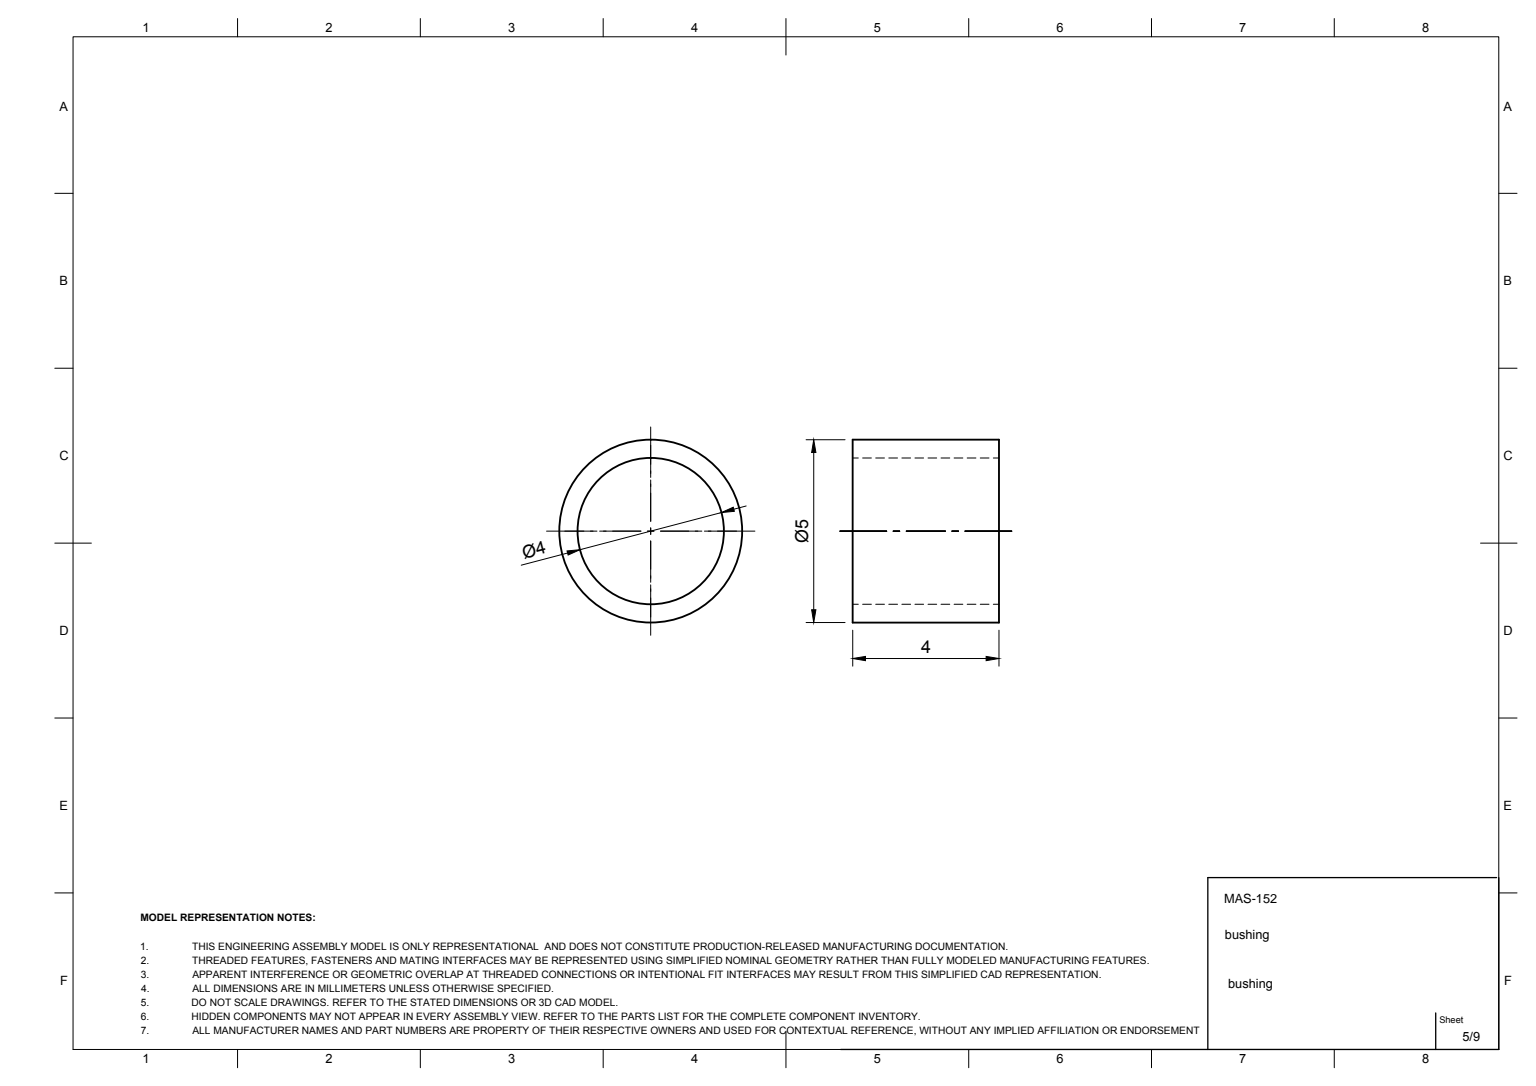
ISO-10303-21;
HEADER;
/* Generated by software containing ST-Developer
 * from STEP Tools, Inc. (www.steptools.com) 
 */

FILE_DESCRIPTION(
/* description */ ('STEP AP214'),
/* implementation_level */ '2;1');

FILE_NAME(
/* name */ 'bushing.step',
/* time_stamp */ '2026-11-04T19:18:53-08:00',
/* author */ (''),
/* organization */ (''),
/* preprocessor_version */ 'ST-DEVELOPER v20.2',
/* originating_system */ 'Autodesk Translation Framework v15.17.0.0',
/* authorisation */ '');

FILE_SCHEMA (('AUTOMOTIVE_DESIGN { 1 0 10303 214 3 1 1 }'));
ENDSEC;

DATA;
#10=MECHANICAL_DESIGN_GEOMETRIC_PRESENTATION_REPRESENTATION('',(#78),#5942);
#64=SHAPE_REPRESENTATION_RELATIONSHIP('SRR','None',#5975,#71);
#71=ADVANCED_BREP_SHAPE_REPRESENTATION('',(#85),#5935);
#78=STYLED_ITEM('',(#6019),#85);
#85=MANIFOLD_SOLID_BREP('Body1',#925);
#92=FACE_BOUND('',#197,.T.);
#93=FACE_BOUND('',#199,.T.);
#100=PLANE('',#1018);
#101=PLANE('',#1019);
#140=FACE_OUTER_BOUND('',#194,.T.);
#141=FACE_OUTER_BOUND('',#195,.T.);
#142=FACE_OUTER_BOUND('',#196,.T.);
#143=FACE_OUTER_BOUND('',#198,.T.);
#194=EDGE_LOOP('',(#634,#635,#636,#637));
#195=EDGE_LOOP('',(#638,#639,#640,#641));
#196=EDGE_LOOP('',(#642));
#197=EDGE_LOOP('',(#643));
#198=EDGE_LOOP('',(#644));
#199=EDGE_LOOP('',(#645));
#256=LINE('',#1397,#334);
#257=LINE('',#1403,#335);
#334=VECTOR('',#1119,2.);
#335=VECTOR('',#1126,2.5);
#412=CIRCLE('',#1013,2.);
#413=CIRCLE('',#1014,2.);
#414=CIRCLE('',#1016,2.5);
#415=CIRCLE('',#1017,2.5);
#444=VERTEX_POINT('',#1394);
#445=VERTEX_POINT('',#1396);
#446=VERTEX_POINT('',#1400);
#447=VERTEX_POINT('',#1402);
#520=EDGE_CURVE('',#444,#444,#412,.T.);
#521=EDGE_CURVE('',#444,#445,#256,.T.);
#522=EDGE_CURVE('',#445,#445,#413,.T.);
#523=EDGE_CURVE('',#446,#446,#414,.T.);
#524=EDGE_CURVE('',#446,#447,#257,.T.);
#525=EDGE_CURVE('',#447,#447,#415,.T.);
#634=ORIENTED_EDGE('',*,*,#520,.T.);
#635=ORIENTED_EDGE('',*,*,#521,.T.);
#636=ORIENTED_EDGE('',*,*,#522,.F.);
#637=ORIENTED_EDGE('',*,*,#521,.F.);
#638=ORIENTED_EDGE('',*,*,#523,.T.);
#639=ORIENTED_EDGE('',*,*,#524,.T.);
#640=ORIENTED_EDGE('',*,*,#525,.F.);
#641=ORIENTED_EDGE('',*,*,#524,.F.);
#642=ORIENTED_EDGE('',*,*,#525,.T.);
#643=ORIENTED_EDGE('',*,*,#520,.F.);
#644=ORIENTED_EDGE('',*,*,#523,.F.);
#645=ORIENTED_EDGE('',*,*,#522,.T.);
#862=CYLINDRICAL_SURFACE('',#1012,2.);
#863=CYLINDRICAL_SURFACE('',#1015,2.5);
#871=ADVANCED_FACE('',(#140),#862,.F.);
#872=ADVANCED_FACE('',(#141),#863,.T.);
#873=ADVANCED_FACE('',(#142,#92),#100,.T.);
#874=ADVANCED_FACE('',(#143,#93),#101,.F.);
#925=CLOSED_SHELL('',(#871,#872,#873,#874));
#1011=AXIS2_PLACEMENT_3D('',#1392,#1113,#1114);
#1012=AXIS2_PLACEMENT_3D('',#1393,#1115,#1116);
#1013=AXIS2_PLACEMENT_3D('',#1395,#1117,#1118);
#1014=AXIS2_PLACEMENT_3D('',#1398,#1120,#1121);
#1015=AXIS2_PLACEMENT_3D('',#1399,#1122,#1123);
#1016=AXIS2_PLACEMENT_3D('',#1401,#1124,#1125);
#1017=AXIS2_PLACEMENT_3D('',#1404,#1127,#1128);
#1018=AXIS2_PLACEMENT_3D('',#1405,#1129,#1130);
#1019=AXIS2_PLACEMENT_3D('',#1406,#1131,#1132);
#1113=DIRECTION('axis',(0.,0.,1.));
#1114=DIRECTION('refdir',(1.,0.,0.));
#1115=DIRECTION('center_axis',(0.,0.,-1.));
#1116=DIRECTION('ref_axis',(-1.,0.,0.));
#1117=DIRECTION('center_axis',(0.,0.,1.));
#1118=DIRECTION('ref_axis',(1.,0.,0.));
#1119=DIRECTION('',(0.,0.,-1.));
#1120=DIRECTION('center_axis',(0.,0.,1.));
#1121=DIRECTION('ref_axis',(1.,0.,0.));
#1122=DIRECTION('center_axis',(0.,0.,-1.));
#1123=DIRECTION('ref_axis',(-1.,0.,0.));
#1124=DIRECTION('center_axis',(0.,0.,1.));
#1125=DIRECTION('ref_axis',(1.,0.,0.));
#1126=DIRECTION('',(0.,0.,1.));
#1127=DIRECTION('center_axis',(0.,0.,1.));
#1128=DIRECTION('ref_axis',(1.,0.,0.));
#1129=DIRECTION('center_axis',(0.,0.,1.));
#1130=DIRECTION('ref_axis',(1.,0.,0.));
#1131=DIRECTION('center_axis',(0.,0.,1.));
#1132=DIRECTION('ref_axis',(1.,0.,0.));
#1392=CARTESIAN_POINT('',(0.,0.,0.));
#1393=CARTESIAN_POINT('Origin',(0.,0.,2.));
#1394=CARTESIAN_POINT('',(2.,-2.44929359829471E-16,2.));
#1395=CARTESIAN_POINT('Origin',(0.,0.,2.));
#1396=CARTESIAN_POINT('',(2.,-2.44929359829471E-16,-2.));
#1397=CARTESIAN_POINT('',(2.,-2.44929359829471E-16,2.));
#1398=CARTESIAN_POINT('Origin',(0.,0.,-2.));
#1399=CARTESIAN_POINT('Origin',(0.,0.,2.));
#1400=CARTESIAN_POINT('',(2.5,-3.06161699786838E-16,-2.));
#1401=CARTESIAN_POINT('Origin',(0.,0.,-2.));
#1402=CARTESIAN_POINT('',(2.5,-3.06161699786838E-16,2.));
#1403=CARTESIAN_POINT('',(2.5,-3.06161699786838E-16,2.));
#1404=CARTESIAN_POINT('Origin',(0.,0.,2.));
#1405=CARTESIAN_POINT('Origin',(0.,0.,2.));
#1406=CARTESIAN_POINT('Origin',(0.,0.,-2.));
#5926=UNCERTAINTY_MEASURE_WITH_UNIT(LENGTH_MEASURE(0.01),#5943,
'DISTANCE_ACCURACY_VALUE',
'Maximum model space distance between geometric entities at asserted c
onnectivities');
#5933=UNCERTAINTY_MEASURE_WITH_UNIT(LENGTH_MEASURE(0.01),#5943,
'DISTANCE_ACCURACY_VALUE',
'Maximum model space distance between geometric entities at asserted c
onnectivities');
#5935=(
GEOMETRIC_REPRESENTATION_CONTEXT(3)
GLOBAL_UNCERTAINTY_ASSIGNED_CONTEXT((#5926))
GLOBAL_UNIT_ASSIGNED_CONTEXT((#5943,#5945,#5946))
REPRESENTATION_CONTEXT('','3D')
);
#5942=(
GEOMETRIC_REPRESENTATION_CONTEXT(3)
GLOBAL_UNCERTAINTY_ASSIGNED_CONTEXT((#5933))
GLOBAL_UNIT_ASSIGNED_CONTEXT((#5943,#5945,#5946))
REPRESENTATION_CONTEXT('','3D')
);
#5943=(
LENGTH_UNIT()
NAMED_UNIT(*)
SI_UNIT(.MILLI.,.METRE.)
);
#5945=(
NAMED_UNIT(*)
PLANE_ANGLE_UNIT()
SI_UNIT($,.RADIAN.)
);
#5946=(
NAMED_UNIT(*)
SI_UNIT($,.STERADIAN.)
SOLID_ANGLE_UNIT()
);
#5948=SHAPE_DEFINITION_REPRESENTATION(#5956,#5975);
#5956=PRODUCT_DEFINITION_SHAPE('',$,#5984);
#5975=SHAPE_REPRESENTATION('',(#1011),#5935);
#5982=PRODUCT_DEFINITION_CONTEXT('part definition',#6008,'design');
#5984=PRODUCT_DEFINITION('bushing','bushing',#5992,#5982);
#5992=PRODUCT_DEFINITION_FORMATION('',$,#6011);
#6008=APPLICATION_CONTEXT(
'Core Data for Automotive Mechanical Design Process');
#6009=PRODUCT_CONTEXT('part definition',#6008,'mechanical');
#6011=PRODUCT('bushing','bushing',$,(#6009));
#6019=PRESENTATION_STYLE_ASSIGNMENT((#6025));
#6025=SURFACE_STYLE_USAGE(.BOTH.,#6031);
#6031=SURFACE_SIDE_STYLE('',(#6037));
#6037=SURFACE_STYLE_FILL_AREA(#6043);
#6043=FILL_AREA_STYLE('Opaque(227,224,212)',(#6049));
#6049=FILL_AREA_STYLE_COLOUR('Opaque(227,224,212)',#6055);
#6055=COLOUR_RGB('Opaque(227,224,212)',0.890196078431372,0.87843137254902,
0.831372549019608);
ENDSEC;
END-ISO-10303-21;
